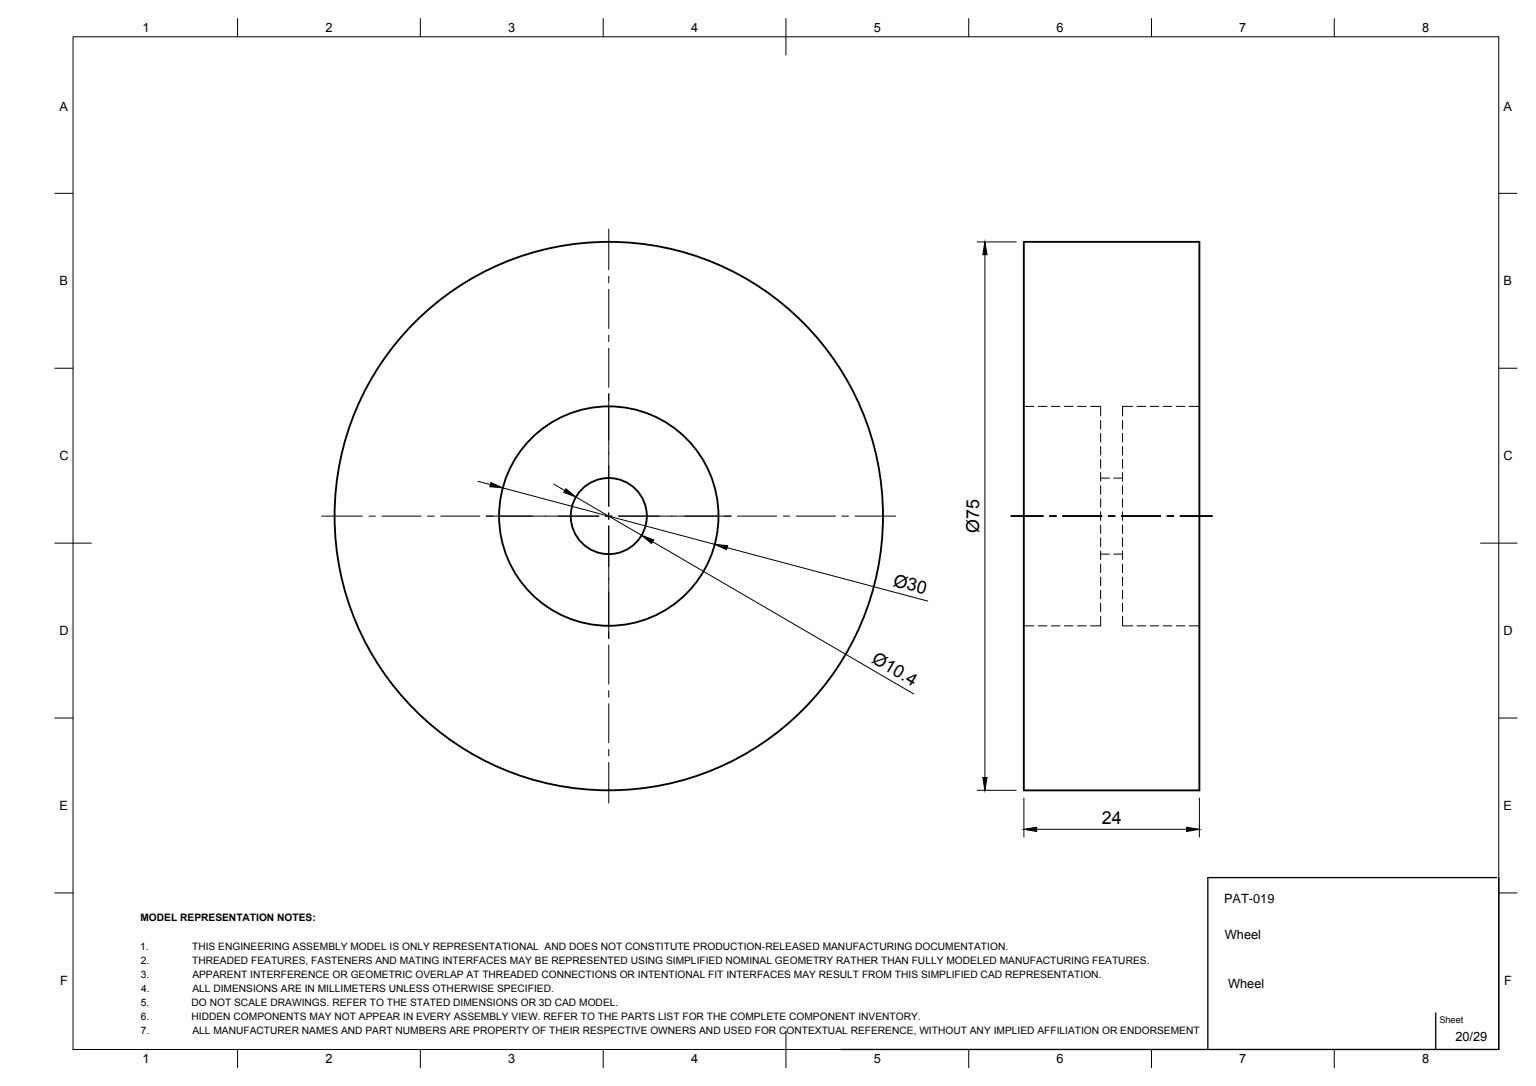
ISO-10303-21;
HEADER;
/* Generated by software containing ST-Developer
 * from STEP Tools, Inc. (www.steptools.com) 
 */

FILE_DESCRIPTION(
/* description */ ('Caster wheel assembly'),
/* implementation_level */ '2;1');

FILE_NAME(
/* name */ 'Wheel.step',
/* time_stamp */ '2026-10-28T03:23:56-07:00',
/* author */ (''),
/* organization */ (''),
/* preprocessor_version */ 'ST-DEVELOPER v20.2',
/* originating_system */ 'Autodesk Translation Framework v15.17.0.0',
/* authorisation */ '');

FILE_SCHEMA (('AUTOMOTIVE_DESIGN { 1 0 10303 214 3 1 1 }'));
ENDSEC;

DATA;
#10=MECHANICAL_DESIGN_GEOMETRIC_PRESENTATION_REPRESENTATION('',(#236),#5385);
#192=SHAPE_REPRESENTATION_RELATIONSHIP('SRR','None',#5489,#214);
#214=ADVANCED_BREP_SHAPE_REPRESENTATION('',(#265),#5376);
#236=STYLED_ITEM('',(#5686),#265);
#265=MANIFOLD_SOLID_BREP('Body1',#2664);
#316=FACE_BOUND('',#727,.T.);
#317=FACE_BOUND('',#730,.T.);
#318=FACE_BOUND('',#734,.T.);
#319=FACE_BOUND('',#736,.T.);
#396=PLANE('',#3131);
#397=PLANE('',#3136);
#398=PLANE('',#3142);
#399=PLANE('',#3143);
#522=FACE_OUTER_BOUND('',#725,.T.);
#523=FACE_OUTER_BOUND('',#726,.T.);
#524=FACE_OUTER_BOUND('',#728,.T.);
#525=FACE_OUTER_BOUND('',#729,.T.);
#526=FACE_OUTER_BOUND('',#731,.T.);
#527=FACE_OUTER_BOUND('',#732,.T.);
#528=FACE_OUTER_BOUND('',#733,.T.);
#529=FACE_OUTER_BOUND('',#735,.T.);
#725=EDGE_LOOP('',(#2168,#2169,#2170,#2171));
#726=EDGE_LOOP('',(#2172));
#727=EDGE_LOOP('',(#2173));
#728=EDGE_LOOP('',(#2174,#2175,#2176,#2177));
#729=EDGE_LOOP('',(#2178));
#730=EDGE_LOOP('',(#2179));
#731=EDGE_LOOP('',(#2180,#2181,#2182,#2183));
#732=EDGE_LOOP('',(#2184,#2185,#2186,#2187));
#733=EDGE_LOOP('',(#2188));
#734=EDGE_LOOP('',(#2189));
#735=EDGE_LOOP('',(#2190));
#736=EDGE_LOOP('',(#2191));
#919=LINE('',#4682,#1053);
#920=LINE('',#4691,#1054);
#921=LINE('',#4697,#1055);
#922=LINE('',#4702,#1056);
#1053=VECTOR('',#3828,1.5);
#1054=VECTOR('',#3839,1.5);
#1055=VECTOR('',#3848,0.52);
#1056=VECTOR('',#3853,3.75);
#1148=CIRCLE('',#3129,1.5);
#1149=CIRCLE('',#3130,1.5);
#1150=CIRCLE('',#3132,0.52);
#1151=CIRCLE('',#3134,1.5);
#1152=CIRCLE('',#3135,1.5);
#1153=CIRCLE('',#3137,0.52);
#1154=CIRCLE('',#3140,3.75);
#1155=CIRCLE('',#3141,3.75);
#1363=VERTEX_POINT('',#4679);
#1364=VERTEX_POINT('',#4681);
#1365=VERTEX_POINT('',#4685);
#1366=VERTEX_POINT('',#4688);
#1367=VERTEX_POINT('',#4690);
#1368=VERTEX_POINT('',#4694);
#1369=VERTEX_POINT('',#4699);
#1370=VERTEX_POINT('',#4701);
#1652=EDGE_CURVE('',#1363,#1363,#1148,.T.);
#1653=EDGE_CURVE('',#1363,#1364,#919,.T.);
#1654=EDGE_CURVE('',#1364,#1364,#1149,.T.);
#1655=EDGE_CURVE('',#1365,#1365,#1150,.T.);
#1656=EDGE_CURVE('',#1366,#1366,#1151,.T.);
#1657=EDGE_CURVE('',#1366,#1367,#920,.T.);
#1658=EDGE_CURVE('',#1367,#1367,#1152,.T.);
#1659=EDGE_CURVE('',#1368,#1368,#1153,.T.);
#1660=EDGE_CURVE('',#1365,#1368,#921,.T.);
#1661=EDGE_CURVE('',#1369,#1369,#1154,.T.);
#1662=EDGE_CURVE('',#1369,#1370,#922,.T.);
#1663=EDGE_CURVE('',#1370,#1370,#1155,.T.);
#2168=ORIENTED_EDGE('',*,*,#1652,.F.);
#2169=ORIENTED_EDGE('',*,*,#1653,.T.);
#2170=ORIENTED_EDGE('',*,*,#1654,.F.);
#2171=ORIENTED_EDGE('',*,*,#1653,.F.);
#2172=ORIENTED_EDGE('',*,*,#1652,.T.);
#2173=ORIENTED_EDGE('',*,*,#1655,.F.);
#2174=ORIENTED_EDGE('',*,*,#1656,.F.);
#2175=ORIENTED_EDGE('',*,*,#1657,.T.);
#2176=ORIENTED_EDGE('',*,*,#1658,.T.);
#2177=ORIENTED_EDGE('',*,*,#1657,.F.);
#2178=ORIENTED_EDGE('',*,*,#1658,.F.);
#2179=ORIENTED_EDGE('',*,*,#1659,.F.);
#2180=ORIENTED_EDGE('',*,*,#1655,.T.);
#2181=ORIENTED_EDGE('',*,*,#1660,.T.);
#2182=ORIENTED_EDGE('',*,*,#1659,.T.);
#2183=ORIENTED_EDGE('',*,*,#1660,.F.);
#2184=ORIENTED_EDGE('',*,*,#1661,.F.);
#2185=ORIENTED_EDGE('',*,*,#1662,.T.);
#2186=ORIENTED_EDGE('',*,*,#1663,.T.);
#2187=ORIENTED_EDGE('',*,*,#1662,.F.);
#2188=ORIENTED_EDGE('',*,*,#1661,.T.);
#2189=ORIENTED_EDGE('',*,*,#1654,.T.);
#2190=ORIENTED_EDGE('',*,*,#1663,.F.);
#2191=ORIENTED_EDGE('',*,*,#1656,.T.);
#2461=CYLINDRICAL_SURFACE('',#3128,1.5);
#2462=CYLINDRICAL_SURFACE('',#3133,1.5);
#2463=CYLINDRICAL_SURFACE('',#3138,0.52);
#2464=CYLINDRICAL_SURFACE('',#3139,3.75);
#2582=ADVANCED_FACE('',(#522),#2461,.F.);
#2583=ADVANCED_FACE('',(#523,#316),#396,.T.);
#2584=ADVANCED_FACE('',(#524),#2462,.F.);
#2585=ADVANCED_FACE('',(#525,#317),#397,.F.);
#2586=ADVANCED_FACE('',(#526),#2463,.F.);
#2587=ADVANCED_FACE('',(#527),#2464,.T.);
#2588=ADVANCED_FACE('',(#528,#318),#398,.T.);
#2589=ADVANCED_FACE('',(#529,#319),#399,.F.);
#2664=CLOSED_SHELL('',(#2582,#2583,#2584,#2585,#2586,#2587,#2588,#2589));
#3127=AXIS2_PLACEMENT_3D('',#4677,#3822,#3823);
#3128=AXIS2_PLACEMENT_3D('',#4678,#3824,#3825);
#3129=AXIS2_PLACEMENT_3D('',#4680,#3826,#3827);
#3130=AXIS2_PLACEMENT_3D('',#4683,#3829,#3830);
#3131=AXIS2_PLACEMENT_3D('',#4684,#3831,#3832);
#3132=AXIS2_PLACEMENT_3D('',#4686,#3833,#3834);
#3133=AXIS2_PLACEMENT_3D('',#4687,#3835,#3836);
#3134=AXIS2_PLACEMENT_3D('',#4689,#3837,#3838);
#3135=AXIS2_PLACEMENT_3D('',#4692,#3840,#3841);
#3136=AXIS2_PLACEMENT_3D('',#4693,#3842,#3843);
#3137=AXIS2_PLACEMENT_3D('',#4695,#3844,#3845);
#3138=AXIS2_PLACEMENT_3D('',#4696,#3846,#3847);
#3139=AXIS2_PLACEMENT_3D('',#4698,#3849,#3850);
#3140=AXIS2_PLACEMENT_3D('',#4700,#3851,#3852);
#3141=AXIS2_PLACEMENT_3D('',#4703,#3854,#3855);
#3142=AXIS2_PLACEMENT_3D('',#4704,#3856,#3857);
#3143=AXIS2_PLACEMENT_3D('',#4705,#3858,#3859);
#3822=DIRECTION('axis',(0.,0.,1.));
#3823=DIRECTION('refdir',(1.,0.,0.));
#3824=DIRECTION('center_axis',(0.,1.,0.));
#3825=DIRECTION('ref_axis',(1.,0.,0.));
#3826=DIRECTION('center_axis',(0.,1.,0.));
#3827=DIRECTION('ref_axis',(1.,0.,0.));
#3828=DIRECTION('',(0.,1.,0.));
#3829=DIRECTION('center_axis',(0.,-1.,0.));
#3830=DIRECTION('ref_axis',(1.,0.,0.));
#3831=DIRECTION('center_axis',(0.,1.,0.));
#3832=DIRECTION('ref_axis',(1.,0.,0.));
#3833=DIRECTION('center_axis',(0.,1.,0.));
#3834=DIRECTION('ref_axis',(1.,0.,0.));
#3835=DIRECTION('center_axis',(0.,1.,0.));
#3836=DIRECTION('ref_axis',(1.,0.,0.));
#3837=DIRECTION('center_axis',(0.,1.,0.));
#3838=DIRECTION('ref_axis',(1.,0.,0.));
#3839=DIRECTION('',(0.,1.,0.));
#3840=DIRECTION('center_axis',(0.,1.,0.));
#3841=DIRECTION('ref_axis',(1.,0.,0.));
#3842=DIRECTION('center_axis',(0.,1.,0.));
#3843=DIRECTION('ref_axis',(1.,0.,0.));
#3844=DIRECTION('center_axis',(0.,-1.,0.));
#3845=DIRECTION('ref_axis',(1.,0.,0.));
#3846=DIRECTION('center_axis',(0.,1.,0.));
#3847=DIRECTION('ref_axis',(1.,0.,0.));
#3848=DIRECTION('',(0.,-1.,0.));
#3849=DIRECTION('center_axis',(0.,1.,0.));
#3850=DIRECTION('ref_axis',(1.,0.,0.));
#3851=DIRECTION('center_axis',(0.,1.,0.));
#3852=DIRECTION('ref_axis',(1.,0.,0.));
#3853=DIRECTION('',(0.,-1.,0.));
#3854=DIRECTION('center_axis',(0.,1.,0.));
#3855=DIRECTION('ref_axis',(1.,0.,0.));
#3856=DIRECTION('center_axis',(0.,1.,0.));
#3857=DIRECTION('ref_axis',(1.,0.,0.));
#3858=DIRECTION('center_axis',(0.,1.,0.));
#3859=DIRECTION('ref_axis',(1.,0.,0.));
#4677=CARTESIAN_POINT('',(0.,0.,0.));
#4678=CARTESIAN_POINT('Origin',(0.,0.15,4.));
#4679=CARTESIAN_POINT('',(-1.5,0.15,4.));
#4680=CARTESIAN_POINT('Origin',(0.,0.15,4.));
#4681=CARTESIAN_POINT('',(-1.5,1.2,4.));
#4682=CARTESIAN_POINT('',(-1.5,0.15,4.));
#4683=CARTESIAN_POINT('Origin',(0.,1.2,4.));
#4684=CARTESIAN_POINT('Origin',(0.,0.15,4.));
#4685=CARTESIAN_POINT('',(-0.52,0.15,4.));
#4686=CARTESIAN_POINT('Origin',(0.,0.15,4.));
#4687=CARTESIAN_POINT('Origin',(0.,-1.3,4.));
#4688=CARTESIAN_POINT('',(-1.5,-1.2,4.));
#4689=CARTESIAN_POINT('Origin',(0.,-1.2,4.));
#4690=CARTESIAN_POINT('',(-1.5,-0.15,4.));
#4691=CARTESIAN_POINT('',(-1.5,-1.3,4.));
#4692=CARTESIAN_POINT('Origin',(0.,-0.15,4.));
#4693=CARTESIAN_POINT('Origin',(0.,-0.15,4.));
#4694=CARTESIAN_POINT('',(-0.52,-0.15,4.));
#4695=CARTESIAN_POINT('Origin',(0.,-0.15,4.));
#4696=CARTESIAN_POINT('Origin',(0.,-1.2,4.));
#4697=CARTESIAN_POINT('',(-0.52,-1.2,4.));
#4698=CARTESIAN_POINT('Origin',(0.,-1.2,4.));
#4699=CARTESIAN_POINT('',(-3.75,1.2,4.));
#4700=CARTESIAN_POINT('Origin',(0.,1.2,4.));
#4701=CARTESIAN_POINT('',(-3.75,-1.2,4.));
#4702=CARTESIAN_POINT('',(-3.75,-1.2,4.));
#4703=CARTESIAN_POINT('Origin',(0.,-1.2,4.));
#4704=CARTESIAN_POINT('Origin',(0.,1.2,4.));
#4705=CARTESIAN_POINT('Origin',(0.,-1.2,4.));
#5348=UNCERTAINTY_MEASURE_WITH_UNIT(LENGTH_MEASURE(0.001),#5386,
'DISTANCE_ACCURACY_VALUE',
'Maximum model space distance between geometric entities at asserted c
onnectivities');
#5357=UNCERTAINTY_MEASURE_WITH_UNIT(LENGTH_MEASURE(0.001),#5386,
'DISTANCE_ACCURACY_VALUE',
'Maximum model space distance between geometric entities at asserted c
onnectivities');
#5376=(
GEOMETRIC_REPRESENTATION_CONTEXT(3)
GLOBAL_UNCERTAINTY_ASSIGNED_CONTEXT((#5348))
GLOBAL_UNIT_ASSIGNED_CONTEXT((#5386,#5388,#5389))
REPRESENTATION_CONTEXT('','3D')
);
#5385=(
GEOMETRIC_REPRESENTATION_CONTEXT(3)
GLOBAL_UNCERTAINTY_ASSIGNED_CONTEXT((#5357))
GLOBAL_UNIT_ASSIGNED_CONTEXT((#5386,#5388,#5389))
REPRESENTATION_CONTEXT('','3D')
);
#5386=(
LENGTH_UNIT()
NAMED_UNIT(*)
SI_UNIT(.CENTI.,.METRE.)
);
#5388=(
NAMED_UNIT(*)
PLANE_ANGLE_UNIT()
SI_UNIT($,.RADIAN.)
);
#5389=(
NAMED_UNIT(*)
SI_UNIT($,.STERADIAN.)
SOLID_ANGLE_UNIT()
);
#5408=SHAPE_DEFINITION_REPRESENTATION(#5449,#5489);
#5449=PRODUCT_DEFINITION_SHAPE('',$,#5517);
#5489=SHAPE_REPRESENTATION('',(#3127),#5376);
#5498=PRODUCT_DEFINITION_CONTEXT('part definition',#5581,'design');
#5517=PRODUCT_DEFINITION('Wheel','Wheel',#5544,#5498);
#5544=PRODUCT_DEFINITION_FORMATION('',$,#5601);
#5581=APPLICATION_CONTEXT(
'Core Data for Automotive Mechanical Design Process');
#5582=PRODUCT_CONTEXT('part definition',#5581,'mechanical');
#5601=PRODUCT('Wheel','Wheel','Wheel',(#5582));
#5680=COLOUR_RGB('Off White',0.89,0.88,0.83);
#5681=FILL_AREA_STYLE_COLOUR('',#5680);
#5682=FILL_AREA_STYLE('',(#5681));
#5683=SURFACE_STYLE_FILL_AREA(#5682);
#5684=SURFACE_SIDE_STYLE('',(#5683));
#5685=SURFACE_STYLE_USAGE(.BOTH.,#5684);
#5686=PRESENTATION_STYLE_ASSIGNMENT((#5685));
ENDSEC;
END-ISO-10303-21;
